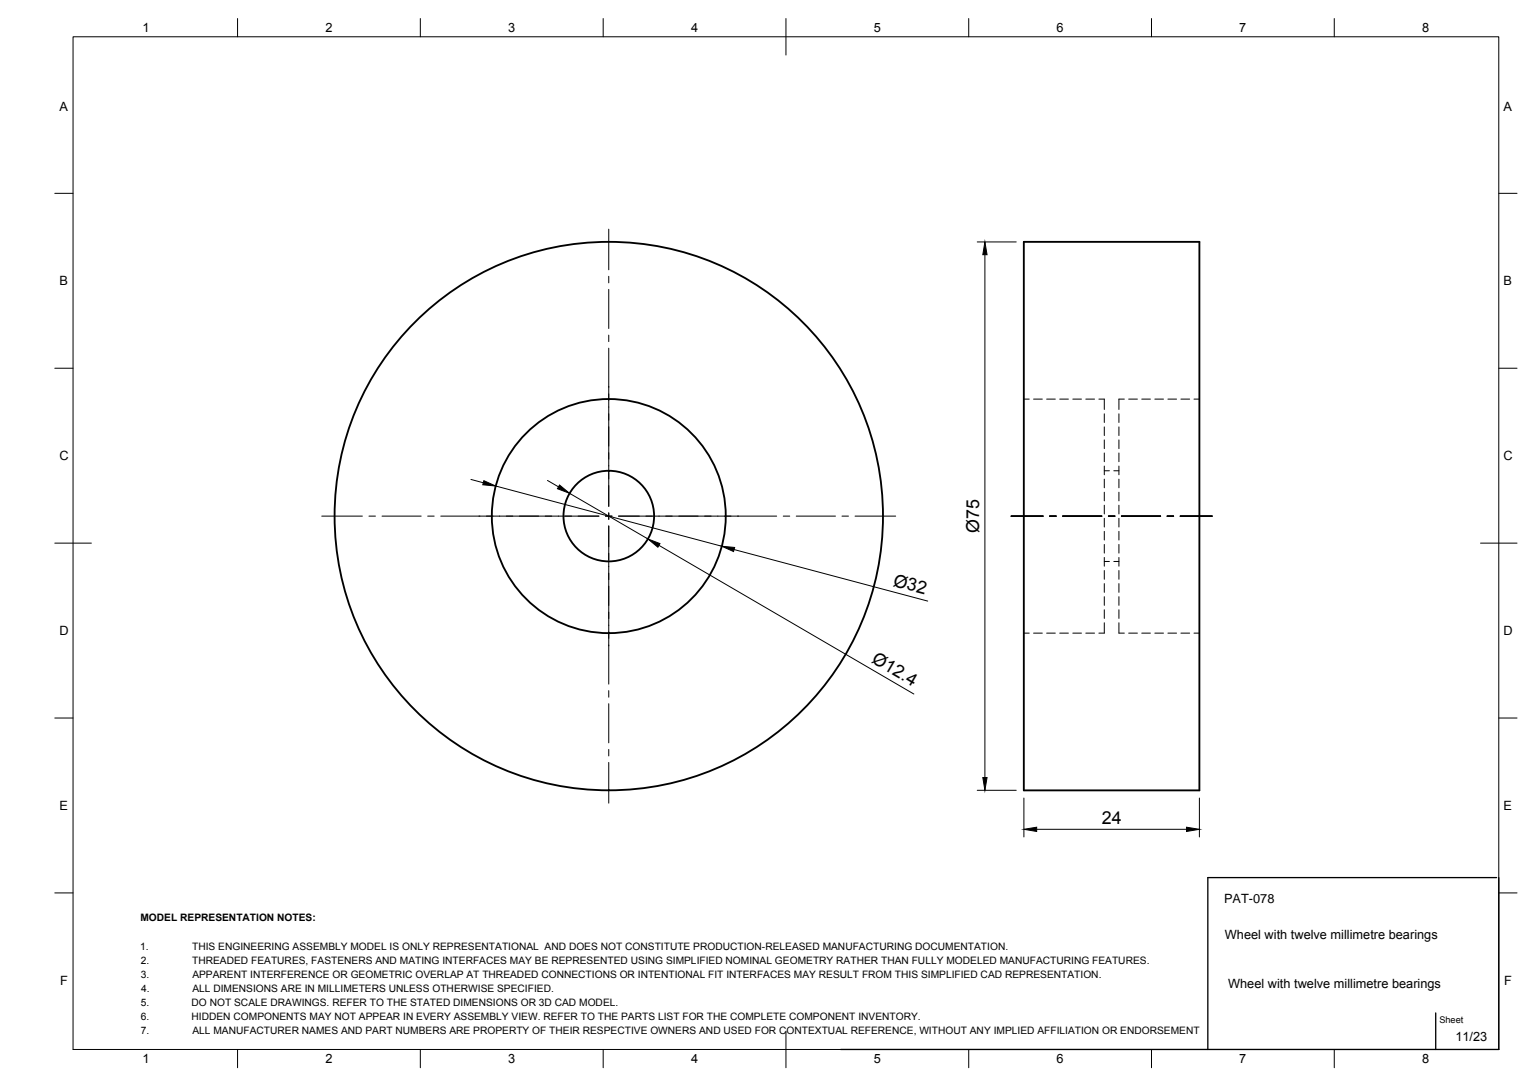
ISO-10303-21;
HEADER;
/* Generated by software containing ST-Developer
 * from STEP Tools, Inc. (www.steptools.com) 
 */

FILE_DESCRIPTION(
/* description */ ('Pedal-braked fixed caster'),
/* implementation_level */ '2;1');

FILE_NAME(
/* name */ 'Wheel with twelve millimetre bearings.step',
/* time_stamp */ '2026-10-28T03:26:52-07:00',
/* author */ (''),
/* organization */ (''),
/* preprocessor_version */ 'ST-DEVELOPER v20.2',
/* originating_system */ 'Autodesk Translation Framework v15.17.0.0',
/* authorisation */ '');

FILE_SCHEMA (('AUTOMOTIVE_DESIGN { 1 0 10303 214 3 1 1 }'));
ENDSEC;

DATA;
#10=MECHANICAL_DESIGN_GEOMETRIC_PRESENTATION_REPRESENTATION('',(#214),#5734);
#180=SHAPE_REPRESENTATION_RELATIONSHIP('SRR','None',#5819,#197);
#197=ADVANCED_BREP_SHAPE_REPRESENTATION('',(#237),#5723);
#214=STYLED_ITEM('',(#5984),#237);
#237=MANIFOLD_SOLID_BREP('Body1',#2996);
#274=CYLINDRICAL_SURFACE('',#3371,1.6);
#275=CYLINDRICAL_SURFACE('',#3376,1.6);
#276=CYLINDRICAL_SURFACE('',#3381,0.62);
#277=CYLINDRICAL_SURFACE('',#3382,3.75);
#323=FACE_BOUND('',#784,.T.);
#324=FACE_BOUND('',#787,.T.);
#325=FACE_BOUND('',#791,.T.);
#326=FACE_BOUND('',#793,.T.);
#389=CIRCLE('',#3372,1.6);
#390=CIRCLE('',#3373,1.6);
#391=CIRCLE('',#3375,0.62);
#392=CIRCLE('',#3377,1.6);
#393=CIRCLE('',#3378,1.6);
#394=CIRCLE('',#3380,0.62);
#395=CIRCLE('',#3383,3.75);
#396=CIRCLE('',#3384,3.75);
#576=FACE_OUTER_BOUND('',#782,.T.);
#577=FACE_OUTER_BOUND('',#783,.T.);
#578=FACE_OUTER_BOUND('',#785,.T.);
#579=FACE_OUTER_BOUND('',#786,.T.);
#580=FACE_OUTER_BOUND('',#788,.T.);
#581=FACE_OUTER_BOUND('',#789,.T.);
#582=FACE_OUTER_BOUND('',#790,.T.);
#583=FACE_OUTER_BOUND('',#792,.T.);
#782=EDGE_LOOP('',(#2382,#2383,#2384,#2385));
#783=EDGE_LOOP('',(#2386));
#784=EDGE_LOOP('',(#2387));
#785=EDGE_LOOP('',(#2388,#2389,#2390,#2391));
#786=EDGE_LOOP('',(#2392));
#787=EDGE_LOOP('',(#2393));
#788=EDGE_LOOP('',(#2394,#2395,#2396,#2397));
#789=EDGE_LOOP('',(#2398,#2399,#2400,#2401));
#790=EDGE_LOOP('',(#2402));
#791=EDGE_LOOP('',(#2403));
#792=EDGE_LOOP('',(#2404));
#793=EDGE_LOOP('',(#2405));
#1031=LINE('',#5023,#1243);
#1032=LINE('',#5032,#1244);
#1033=LINE('',#5038,#1245);
#1034=LINE('',#5043,#1246);
#1243=VECTOR('',#4061,1.6);
#1244=VECTOR('',#4072,1.6);
#1245=VECTOR('',#4081,0.62);
#1246=VECTOR('',#4086,3.75);
#1446=VERTEX_POINT('',#5020);
#1447=VERTEX_POINT('',#5022);
#1448=VERTEX_POINT('',#5026);
#1449=VERTEX_POINT('',#5029);
#1450=VERTEX_POINT('',#5031);
#1451=VERTEX_POINT('',#5035);
#1452=VERTEX_POINT('',#5040);
#1453=VERTEX_POINT('',#5042);
#1781=EDGE_CURVE('',#1446,#1446,#389,.T.);
#1782=EDGE_CURVE('',#1446,#1447,#1031,.T.);
#1783=EDGE_CURVE('',#1447,#1447,#390,.T.);
#1784=EDGE_CURVE('',#1448,#1448,#391,.T.);
#1785=EDGE_CURVE('',#1449,#1449,#392,.T.);
#1786=EDGE_CURVE('',#1449,#1450,#1032,.T.);
#1787=EDGE_CURVE('',#1450,#1450,#393,.T.);
#1788=EDGE_CURVE('',#1451,#1451,#394,.T.);
#1789=EDGE_CURVE('',#1451,#1448,#1033,.T.);
#1790=EDGE_CURVE('',#1452,#1452,#395,.T.);
#1791=EDGE_CURVE('',#1452,#1453,#1034,.T.);
#1792=EDGE_CURVE('',#1453,#1453,#396,.T.);
#2382=ORIENTED_EDGE('',*,*,#1781,.F.);
#2383=ORIENTED_EDGE('',*,*,#1782,.T.);
#2384=ORIENTED_EDGE('',*,*,#1783,.F.);
#2385=ORIENTED_EDGE('',*,*,#1782,.F.);
#2386=ORIENTED_EDGE('',*,*,#1781,.T.);
#2387=ORIENTED_EDGE('',*,*,#1784,.F.);
#2388=ORIENTED_EDGE('',*,*,#1785,.F.);
#2389=ORIENTED_EDGE('',*,*,#1786,.T.);
#2390=ORIENTED_EDGE('',*,*,#1787,.T.);
#2391=ORIENTED_EDGE('',*,*,#1786,.F.);
#2392=ORIENTED_EDGE('',*,*,#1787,.F.);
#2393=ORIENTED_EDGE('',*,*,#1788,.F.);
#2394=ORIENTED_EDGE('',*,*,#1788,.T.);
#2395=ORIENTED_EDGE('',*,*,#1789,.T.);
#2396=ORIENTED_EDGE('',*,*,#1784,.T.);
#2397=ORIENTED_EDGE('',*,*,#1789,.F.);
#2398=ORIENTED_EDGE('',*,*,#1790,.F.);
#2399=ORIENTED_EDGE('',*,*,#1791,.T.);
#2400=ORIENTED_EDGE('',*,*,#1792,.T.);
#2401=ORIENTED_EDGE('',*,*,#1791,.F.);
#2402=ORIENTED_EDGE('',*,*,#1790,.T.);
#2403=ORIENTED_EDGE('',*,*,#1783,.T.);
#2404=ORIENTED_EDGE('',*,*,#1792,.F.);
#2405=ORIENTED_EDGE('',*,*,#1785,.T.);
#2772=PLANE('',#3374);
#2773=PLANE('',#3379);
#2774=PLANE('',#3385);
#2775=PLANE('',#3386);
#2909=ADVANCED_FACE('',(#576),#274,.F.);
#2910=ADVANCED_FACE('',(#577,#323),#2772,.T.);
#2911=ADVANCED_FACE('',(#578),#275,.F.);
#2912=ADVANCED_FACE('',(#579,#324),#2773,.F.);
#2913=ADVANCED_FACE('',(#580),#276,.F.);
#2914=ADVANCED_FACE('',(#581),#277,.T.);
#2915=ADVANCED_FACE('',(#582,#325),#2774,.T.);
#2916=ADVANCED_FACE('',(#583,#326),#2775,.F.);
#2996=CLOSED_SHELL('',(#2909,#2910,#2911,#2912,#2913,#2914,#2915,#2916));
#3370=AXIS2_PLACEMENT_3D('',#5018,#4055,#4056);
#3371=AXIS2_PLACEMENT_3D('',#5019,#4057,#4058);
#3372=AXIS2_PLACEMENT_3D('',#5021,#4059,#4060);
#3373=AXIS2_PLACEMENT_3D('',#5024,#4062,#4063);
#3374=AXIS2_PLACEMENT_3D('',#5025,#4064,#4065);
#3375=AXIS2_PLACEMENT_3D('',#5027,#4066,#4067);
#3376=AXIS2_PLACEMENT_3D('',#5028,#4068,#4069);
#3377=AXIS2_PLACEMENT_3D('',#5030,#4070,#4071);
#3378=AXIS2_PLACEMENT_3D('',#5033,#4073,#4074);
#3379=AXIS2_PLACEMENT_3D('',#5034,#4075,#4076);
#3380=AXIS2_PLACEMENT_3D('',#5036,#4077,#4078);
#3381=AXIS2_PLACEMENT_3D('',#5037,#4079,#4080);
#3382=AXIS2_PLACEMENT_3D('',#5039,#4082,#4083);
#3383=AXIS2_PLACEMENT_3D('',#5041,#4084,#4085);
#3384=AXIS2_PLACEMENT_3D('',#5044,#4087,#4088);
#3385=AXIS2_PLACEMENT_3D('',#5045,#4089,#4090);
#3386=AXIS2_PLACEMENT_3D('',#5046,#4091,#4092);
#4055=DIRECTION('axis',(0.,0.,1.));
#4056=DIRECTION('refdir',(1.,0.,0.));
#4057=DIRECTION('center_axis',(0.,1.,0.));
#4058=DIRECTION('ref_axis',(1.,0.,0.));
#4059=DIRECTION('center_axis',(0.,1.,0.));
#4060=DIRECTION('ref_axis',(1.,0.,0.));
#4061=DIRECTION('',(0.,1.,0.));
#4062=DIRECTION('center_axis',(0.,-1.,0.));
#4063=DIRECTION('ref_axis',(1.,0.,0.));
#4064=DIRECTION('center_axis',(0.,1.,0.));
#4065=DIRECTION('ref_axis',(1.,0.,0.));
#4066=DIRECTION('center_axis',(0.,1.,0.));
#4067=DIRECTION('ref_axis',(1.,0.,0.));
#4068=DIRECTION('center_axis',(0.,1.,0.));
#4069=DIRECTION('ref_axis',(1.,0.,0.));
#4070=DIRECTION('center_axis',(0.,1.,0.));
#4071=DIRECTION('ref_axis',(1.,0.,0.));
#4072=DIRECTION('',(0.,1.,0.));
#4073=DIRECTION('center_axis',(0.,1.,0.));
#4074=DIRECTION('ref_axis',(1.,0.,0.));
#4075=DIRECTION('center_axis',(0.,1.,0.));
#4076=DIRECTION('ref_axis',(1.,0.,0.));
#4077=DIRECTION('center_axis',(0.,-1.,0.));
#4078=DIRECTION('ref_axis',(1.,0.,0.));
#4079=DIRECTION('center_axis',(0.,1.,0.));
#4080=DIRECTION('ref_axis',(1.,0.,0.));
#4081=DIRECTION('',(0.,1.,0.));
#4082=DIRECTION('center_axis',(0.,1.,0.));
#4083=DIRECTION('ref_axis',(1.,0.,0.));
#4084=DIRECTION('center_axis',(0.,1.,0.));
#4085=DIRECTION('ref_axis',(1.,0.,0.));
#4086=DIRECTION('',(0.,-1.,0.));
#4087=DIRECTION('center_axis',(0.,1.,0.));
#4088=DIRECTION('ref_axis',(1.,0.,0.));
#4089=DIRECTION('center_axis',(0.,1.,0.));
#4090=DIRECTION('ref_axis',(1.,0.,0.));
#4091=DIRECTION('center_axis',(0.,1.,0.));
#4092=DIRECTION('ref_axis',(1.,0.,0.));
#5018=CARTESIAN_POINT('',(0.,0.,0.));
#5019=CARTESIAN_POINT('Origin',(0.,0.1,4.));
#5020=CARTESIAN_POINT('',(-1.6,0.1,4.));
#5021=CARTESIAN_POINT('Origin',(0.,0.1,4.));
#5022=CARTESIAN_POINT('',(-1.6,1.2,4.));
#5023=CARTESIAN_POINT('',(-1.6,0.1,4.));
#5024=CARTESIAN_POINT('Origin',(0.,1.2,4.));
#5025=CARTESIAN_POINT('Origin',(0.,0.1,4.));
#5026=CARTESIAN_POINT('',(-0.62,0.1,4.));
#5027=CARTESIAN_POINT('Origin',(0.,0.1,4.));
#5028=CARTESIAN_POINT('Origin',(0.,-1.3,4.));
#5029=CARTESIAN_POINT('',(-1.6,-1.2,4.));
#5030=CARTESIAN_POINT('Origin',(0.,-1.2,4.));
#5031=CARTESIAN_POINT('',(-1.6,-0.0999999999999999,4.));
#5032=CARTESIAN_POINT('',(-1.6,-1.3,4.));
#5033=CARTESIAN_POINT('Origin',(0.,-0.0999999999999999,4.));
#5034=CARTESIAN_POINT('Origin',(0.,-0.0999999999999999,4.));
#5035=CARTESIAN_POINT('',(-0.62,-0.0999999999999999,4.));
#5036=CARTESIAN_POINT('Origin',(0.,-0.0999999999999999,4.));
#5037=CARTESIAN_POINT('Origin',(0.,-1.3,4.));
#5038=CARTESIAN_POINT('',(-0.62,-1.3,4.));
#5039=CARTESIAN_POINT('Origin',(0.,-1.2,4.));
#5040=CARTESIAN_POINT('',(-3.75,1.2,4.));
#5041=CARTESIAN_POINT('Origin',(0.,1.2,4.));
#5042=CARTESIAN_POINT('',(-3.75,-1.2,4.));
#5043=CARTESIAN_POINT('',(-3.75,-1.2,4.));
#5044=CARTESIAN_POINT('Origin',(0.,-1.2,4.));
#5045=CARTESIAN_POINT('Origin',(0.,1.2,4.));
#5046=CARTESIAN_POINT('Origin',(0.,-1.2,4.));
#5700=UNCERTAINTY_MEASURE_WITH_UNIT(LENGTH_MEASURE(0.001),#5735,
'DISTANCE_ACCURACY_VALUE',
'Maximum model space distance between geometric entities at asserted c
onnectivities');
#5711=UNCERTAINTY_MEASURE_WITH_UNIT(LENGTH_MEASURE(0.001),#5735,
'DISTANCE_ACCURACY_VALUE',
'Maximum model space distance between geometric entities at asserted c
onnectivities');
#5723=(
GEOMETRIC_REPRESENTATION_CONTEXT(3)
GLOBAL_UNCERTAINTY_ASSIGNED_CONTEXT((#5700))
GLOBAL_UNIT_ASSIGNED_CONTEXT((#5735,#5737,#5738))
REPRESENTATION_CONTEXT('','3D')
);
#5734=(
GEOMETRIC_REPRESENTATION_CONTEXT(3)
GLOBAL_UNCERTAINTY_ASSIGNED_CONTEXT((#5711))
GLOBAL_UNIT_ASSIGNED_CONTEXT((#5735,#5737,#5738))
REPRESENTATION_CONTEXT('','3D')
);
#5735=(
LENGTH_UNIT()
NAMED_UNIT(*)
SI_UNIT(.CENTI.,.METRE.)
);
#5737=(
NAMED_UNIT(*)
PLANE_ANGLE_UNIT()
SI_UNIT($,.RADIAN.)
);
#5738=(
NAMED_UNIT(*)
SI_UNIT($,.STERADIAN.)
SOLID_ANGLE_UNIT()
);
#5750=SHAPE_DEFINITION_REPRESENTATION(#5782,#5819);
#5782=PRODUCT_DEFINITION_SHAPE('',$,#5842);
#5819=SHAPE_REPRESENTATION('',(#3370),#5723);
#5830=PRODUCT_DEFINITION_CONTEXT('part definition',#5898,'design');
#5842=PRODUCT_DEFINITION('Wheel with twelve millimetre bearings',
'Wheel with twelve millimetre bearings',#5864,#5830);
#5864=PRODUCT_DEFINITION_FORMATION('',$,#5911);
#5898=APPLICATION_CONTEXT(
'Core Data for Automotive Mechanical Design Process');
#5899=PRODUCT_CONTEXT('part definition',#5898,'mechanical');
#5911=PRODUCT('Wheel with twelve millimetre bearings',
'Wheel with twelve millimetre bearings',
'Wheel with twelve millimetre bearings',(#5899));
#5978=COLOUR_RGB('Grey',0.48,0.52,0.57);
#5979=FILL_AREA_STYLE_COLOUR('',#5978);
#5980=FILL_AREA_STYLE('',(#5979));
#5981=SURFACE_STYLE_FILL_AREA(#5980);
#5982=SURFACE_SIDE_STYLE('',(#5981));
#5983=SURFACE_STYLE_USAGE(.BOTH.,#5982);
#5984=PRESENTATION_STYLE_ASSIGNMENT((#5983));
ENDSEC;
END-ISO-10303-21;
